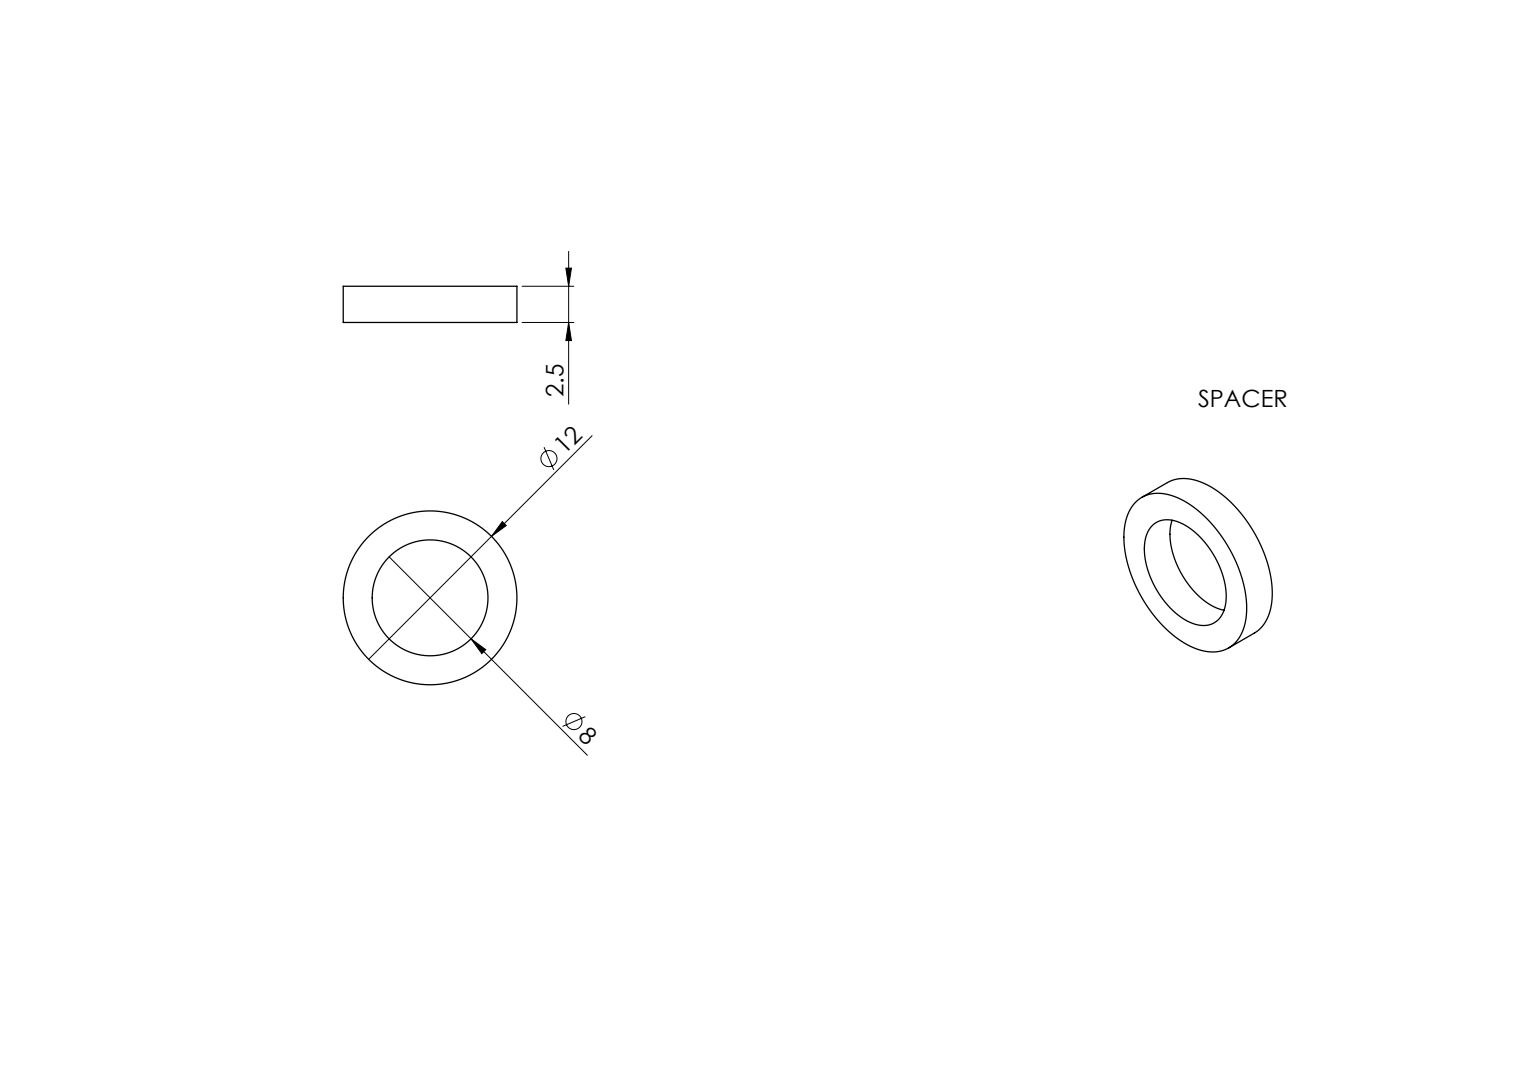
ISO-10303-21;
HEADER;
FILE_DESCRIPTION (('STEP AP214'),
    '1' );
FILE_NAME ('spacer.step',
    '2026-10-31T03:41:51',
    ( '' ),
    ( '' ),
    'SwSTEP 2.0',
    'SolidWorks 2026',
    '' );
FILE_SCHEMA (( 'AUTOMOTIVE_DESIGN' ));
ENDSEC;

DATA;
#19=FACE_OUTER_BOUND ( 'NONE', #11949, .T. ) ;
#42=CYLINDRICAL_SURFACE ( 'NONE', #425, 5.999999999999999112 ) ;
#89=ORIENTED_EDGE ( 'NONE', *, *, #1488, .F. ) ;
#125=PLANE ( 'NONE',  #1631 ) ;
#144=CARTESIAN_POINT ( 'NONE',  ( 0.000000000000000000, 0.000000000000000000, 3.895000000000000462 ) ) ;
#220=CIRCLE ( 'NONE', #8093, 5.999999999999999112 ) ;
#252=ADVANCED_FACE ( 'NONE', ( #6406, #6332 ), #7416, .F. ) ;
#355=ORIENTED_EDGE ( 'NONE', *, *, #8570, .F. ) ;
#402=ORIENTED_EDGE ( 'NONE', *, *, #5553, .T. ) ;
#425=AXIS2_PLACEMENT_3D ( 'NONE', #3589, #8419, #2592 ) ;
#542=PRODUCT_DEFINITION_CONTEXT ( 'detailed design', #8310, 'design' ) ;
#683=AXIS2_PLACEMENT_3D ( 'NONE', #4148, #11052, #7449 ) ;
#791=CARTESIAN_POINT ( 'NONE',  ( 4.000000000000000000, 4.898587196589412829E-16, 3.895000000000000462 ) ) ;
#805=AXIS2_PLACEMENT_3D ( 'NONE', #9265, #4731, #5810 ) ;
#1155=AXIS2_PLACEMENT_3D ( 'NONE', #2651, #6177, #5122 ) ;
#1175=CARTESIAN_POINT ( 'NONE',  ( -5.999999999999999112, 0.000000000000000000, 1.395000000000000462 ) ) ;
#1312=ORIENTED_EDGE ( 'NONE', *, *, #4480, .F. ) ;
#1357=DIRECTION ( 'NONE',  ( -0.000000000000000000, -0.000000000000000000, -1.000000000000000000 ) ) ;
#1376=AXIS2_PLACEMENT_3D ( 'NONE', #7353, #6187, #9640 ) ;
#1391=DIRECTION ( 'NONE',  ( 0.000000000000000000, 0.000000000000000000, -1.000000000000000000 ) ) ;
#1443=LINE ( 'NONE', #3512, #4366 ) ;
#1488=EDGE_CURVE ( 'NONE', #5963, #15052, #13663, .T. ) ;
#1631=AXIS2_PLACEMENT_3D ( 'NONE', #2376, #11890, #11748 ) ;
#1634=UNCERTAINTY_MEASURE_WITH_UNIT (LENGTH_MEASURE( 1.000000000000000082E-05 ), #6541, 'distance_accuracy_value', 'NONE');
#1705=SURFACE_STYLE_USAGE ( .BOTH. , #13375 ) ;
#1863=DIRECTION ( 'NONE',  ( -1.000000000000000000, 0.000000000000000000, 0.000000000000000000 ) ) ;
#1949=ADVANCED_FACE ( 'NONE', ( #3680, #12971 ), #125, .T. ) ;
#2053=DIRECTION ( 'NONE',  ( -0.000000000000000000, -0.000000000000000000, -1.000000000000000000 ) ) ;
#2054=EDGE_CURVE ( 'NONE', #3198, #8635, #12421, .T. ) ;
#2071=CARTESIAN_POINT ( 'NONE',  ( 0.000000000000000000, 0.000000000000000000, 3.895000000000000462 ) ) ;
#2078=VERTEX_POINT ( 'NONE', #9893 ) ;
#2095=EDGE_LOOP ( 'NONE', ( #8631, #14510 ) ) ;
#2126=( GEOMETRIC_REPRESENTATION_CONTEXT ( 3 ) GLOBAL_UNCERTAINTY_ASSIGNED_CONTEXT ( ( #1634 ) ) GLOBAL_UNIT_ASSIGNED_CONTEXT ( ( #6541, #8765, #3857 ) ) REPRESENTATION_CONTEXT ( 'NONE', 'WORKASPACE' ) );
#2208=ADVANCED_FACE ( 'NONE', ( #13742 ), #5387, .T. ) ;
#2376=CARTESIAN_POINT ( 'NONE',  ( 0.000000000000000000, 0.000000000000000000, 1.395000000000000462 ) ) ;
#2378=EDGE_CURVE ( 'NONE', #13028, #6156, #2757, .T. ) ;
#2438=DIRECTION ( 'NONE',  ( -1.000000000000000000, 0.000000000000000000, 0.000000000000000000 ) ) ;
#2443=CIRCLE ( 'NONE', #11027, 5.999999999999999112 ) ;
#2592=DIRECTION ( 'NONE',  ( -1.000000000000000000, 0.000000000000000000, 0.000000000000000000 ) ) ;
#2611=MECHANICAL_DESIGN_GEOMETRIC_PRESENTATION_REPRESENTATION('',(#9242),#10950);
#2651=CARTESIAN_POINT ( 'NONE',  ( 0.000000000000000000, 0.000000000000000000, 3.895000000000000462 ) ) ;
#2697=ORIENTED_EDGE ( 'NONE', *, *, #5601, .T. ) ;
#2757=CIRCLE ( 'NONE', #11337, 4.000000000000000000 ) ;
#2777=ORIENTED_EDGE ( 'NONE', *, *, #9895, .F. ) ;
#2831=CIRCLE ( 'NONE', #4804, 5.999999999999999112 ) ;
#2918=AXIS2_PLACEMENT_3D ( 'NONE', #11500, #15210, #6043 ) ;
#3163=CARTESIAN_POINT ( 'NONE',  ( 5.999999999999999112, 7.347880794884118750E-16, 3.895000000000000462 ) ) ;
#3198=VERTEX_POINT ( 'NONE', #11372 ) ;
#3220=CARTESIAN_POINT ( 'NONE',  ( 0.000000000000000000, 0.000000000000000000, 3.895000000000000462 ) ) ;
#3239=EDGE_LOOP ( 'NONE', ( #14240, #4911 ) ) ;
#3355=AXIS2_PLACEMENT_3D ( 'NONE', #5126, #7491, #14495 ) ;
#3480=AXIS2_PLACEMENT_3D ( 'NONE', #3220, #2053, #4220 ) ;
#3512=CARTESIAN_POINT ( 'NONE',  ( -5.999999999999999112, 0.000000000000000000, 3.895000000000000462 ) ) ;
#3589=CARTESIAN_POINT ( 'NONE',  ( 0.000000000000000000, 0.000000000000000000, 3.895000000000000462 ) ) ;
#3619=DIRECTION ( 'NONE',  ( -1.000000000000000000, 0.000000000000000000, 0.000000000000000000 ) ) ;
#3680=FACE_BOUND ( 'NONE', #3239, .T. ) ;
#3746=ORIENTED_EDGE ( 'NONE', *, *, #12567, .F. ) ;
#3857=( NAMED_UNIT ( * ) SI_UNIT ( $, .STERADIAN. ) SOLID_ANGLE_UNIT ( ) );
#4014=ADVANCED_FACE ( 'NONE', ( #19 ), #4890, .F. ) ;
#4057=PRODUCT_CONTEXT ( 'NONE', #14709, 'mechanical' ) ;
#4148=CARTESIAN_POINT ( 'NONE',  ( 0.000000000000000000, 0.000000000000000000, 3.895000000000000462 ) ) ;
#4220=DIRECTION ( 'NONE',  ( -1.000000000000000000, 0.000000000000000000, 0.000000000000000000 ) ) ;
#4282=SHAPE_DEFINITION_REPRESENTATION ( #5673, #13067 ) ;
#4366=VECTOR ( 'NONE', #1357, 1000.000000000000000 ) ;
#4480=EDGE_CURVE ( 'NONE', #2078, #3198, #7919, .T. ) ;
#4731=DIRECTION ( 'NONE',  ( -0.000000000000000000, -0.000000000000000000, -1.000000000000000000 ) ) ;
#4735=VECTOR ( 'NONE', #5693, 1000.000000000000000 ) ;
#4773=ORIENTED_EDGE ( 'NONE', *, *, #8992, .F. ) ;
#4804=AXIS2_PLACEMENT_3D ( 'NONE', #6467, #12381, #1863 ) ;
#4890=CYLINDRICAL_SURFACE ( 'NONE', #805, 4.000000000000000000 ) ;
#4911=ORIENTED_EDGE ( 'NONE', *, *, #2378, .F. ) ;
#5020=( NAMED_UNIT ( * ) PLANE_ANGLE_UNIT ( ) SI_UNIT ( $, .RADIAN. ) );
#5046=ORIENTED_EDGE ( 'NONE', *, *, #2378, .T. ) ;
#5079=CARTESIAN_POINT ( 'NONE',  ( 0.000000000000000000, 0.000000000000000000, 1.395000000000000462 ) ) ;
#5122=DIRECTION ( 'NONE',  ( -1.000000000000000000, 0.000000000000000000, -0.000000000000000000 ) ) ;
#5126=CARTESIAN_POINT ( 'NONE',  ( 0.000000000000000000, 0.000000000000000000, 3.895000000000000462 ) ) ;
#5322=CARTESIAN_POINT ( 'NONE',  ( 0.000000000000000000, 0.000000000000000000, 1.395000000000000462 ) ) ;
#5357=DIRECTION ( 'NONE',  ( -0.000000000000000000, -0.000000000000000000, -1.000000000000000000 ) ) ;
#5387=CYLINDRICAL_SURFACE ( 'NONE', #3480, 5.999999999999999112 ) ;
#5553=EDGE_CURVE ( 'NONE', #8635, #3198, #220, .T. ) ;
#5601=EDGE_CURVE ( 'NONE', #2078, #6712, #2443, .T. ) ;
#5668=DIRECTION ( 'NONE',  ( -0.000000000000000000, -0.000000000000000000, -1.000000000000000000 ) ) ;
#5673=PRODUCT_DEFINITION_SHAPE ( 'NONE', 'NONE',  #11139 ) ;
#5692=DIRECTION ( 'NONE',  ( -1.000000000000000000, 0.000000000000000000, 0.000000000000000000 ) ) ;
#5693=DIRECTION ( 'NONE',  ( -0.000000000000000000, -0.000000000000000000, -1.000000000000000000 ) ) ;
#5743=CARTESIAN_POINT ( 'NONE',  ( -4.000000000000000000, 0.000000000000000000, 1.395000000000000462 ) ) ;
#5810=DIRECTION ( 'NONE',  ( -1.000000000000000000, 0.000000000000000000, 0.000000000000000000 ) ) ;
#5868=ORIENTED_EDGE ( 'NONE', *, *, #9895, .T. ) ;
#5963=VERTEX_POINT ( 'NONE', #7376 ) ;
#6043=DIRECTION ( 'NONE',  ( -1.000000000000000000, 0.000000000000000000, 0.000000000000000000 ) ) ;
#6141=CYLINDRICAL_SURFACE ( 'NONE', #683, 4.000000000000000000 ) ;
#6156=VERTEX_POINT ( 'NONE', #5743 ) ;
#6177=DIRECTION ( 'NONE',  ( 0.000000000000000000, 0.000000000000000000, -1.000000000000000000 ) ) ;
#6187=DIRECTION ( 'NONE',  ( 0.000000000000000000, 0.000000000000000000, 1.000000000000000000 ) ) ;
#6249=( GEOMETRIC_REPRESENTATION_CONTEXT ( 3 ) GLOBAL_UNCERTAINTY_ASSIGNED_CONTEXT ( ( #11534 ) ) GLOBAL_UNIT_ASSIGNED_CONTEXT ( ( #14041, #10436, #7129 ) ) REPRESENTATION_CONTEXT ( 'NONE', 'WORKASPACE' ) );
#6332=FACE_OUTER_BOUND ( 'NONE', #14476, .T. ) ;
#6406=FACE_BOUND ( 'NONE', #2095, .T. ) ;
#6467=CARTESIAN_POINT ( 'NONE',  ( 0.000000000000000000, 0.000000000000000000, 3.895000000000000462 ) ) ;
#6541=( LENGTH_UNIT ( ) NAMED_UNIT ( * ) SI_UNIT ( .MILLI., .METRE. ) );
#6712=VERTEX_POINT ( 'NONE', #7172 ) ;
#6966=CARTESIAN_POINT ( 'NONE',  ( 0.000000000000000000, 0.000000000000000000, 1.395000000000000462 ) ) ;
#7035=AXIS2_PLACEMENT_3D ( 'NONE', #144, #1391, #3619 ) ;
#7040=ADVANCED_FACE ( 'NONE', ( #8513 ), #6141, .F. ) ;
#7129=( NAMED_UNIT ( * ) SI_UNIT ( $, .STERADIAN. ) SOLID_ANGLE_UNIT ( ) );
#7172=CARTESIAN_POINT ( 'NONE',  ( -5.999999999999999112, 0.000000000000000000, 3.895000000000000462 ) ) ;
#7216=CLOSED_SHELL ( 'NONE', ( #4014, #2208, #9609, #252, #1949, #7040 ) ) ;
#7282=CIRCLE ( 'NONE', #3355, 4.000000000000000000 ) ;
#7289=EDGE_CURVE ( 'NONE', #6156, #13028, #8799, .T. ) ;
#7346=ORIENTED_EDGE ( 'NONE', *, *, #2054, .T. ) ;
#7353=CARTESIAN_POINT ( 'NONE',  ( 0.000000000000000000, 0.000000000000000000, 0.000000000000000000 ) ) ;
#7376=CARTESIAN_POINT ( 'NONE',  ( -4.000000000000000000, 0.000000000000000000, 3.895000000000000462 ) ) ;
#7416=PLANE ( 'NONE',  #1155 ) ;
#7449=DIRECTION ( 'NONE',  ( -1.000000000000000000, 0.000000000000000000, 0.000000000000000000 ) ) ;
#7450=DIRECTION ( 'NONE',  ( 0.000000000000000000, 0.000000000000000000, -1.000000000000000000 ) ) ;
#7491=DIRECTION ( 'NONE',  ( 0.000000000000000000, 0.000000000000000000, -1.000000000000000000 ) ) ;
#7623=FILL_AREA_STYLE ('',( #8842 ) ) ;
#7687=DIRECTION ( 'NONE',  ( 0.000000000000000000, 0.000000000000000000, -1.000000000000000000 ) ) ;
#7693=SHAPE_REPRESENTATION_RELATIONSHIP ( 'NONE' , 'NONE' ,  #13067, #8180 ) ;
#7722=STYLED_ITEM('',(#15265),#8383);
#7901=EDGE_LOOP ( 'NONE', ( #9151, #8082, #14292, #9298 ) ) ;
#7919=LINE ( 'NONE', #3163, #4735 ) ;
#8000=EDGE_LOOP ( 'NONE', ( #355, #89, #5868, #8665 ) ) ;
#8082=ORIENTED_EDGE ( 'NONE', *, *, #4480, .T. ) ;
#8093=AXIS2_PLACEMENT_3D ( 'NONE', #5322, #14694, #8837 ) ;
#8180=ADVANCED_BREP_SHAPE_REPRESENTATION ( '', ( #8383, #1376 ), #2126 ) ;
#8310=APPLICATION_CONTEXT ( 'automotive_design' ) ;
#8367=EDGE_LOOP ( 'NONE', ( #1312, #2697, #12223, #12430 ) ) ;
#8383=MANIFOLD_SOLID_BREP ( 'Boss-Extrude1', #7216 ) ;
#8419=DIRECTION ( 'NONE',  ( -0.000000000000000000, -0.000000000000000000, -1.000000000000000000 ) ) ;
#8513=FACE_OUTER_BOUND ( 'NONE', #8000, .T. ) ;
#8541=( LENGTH_UNIT ( ) NAMED_UNIT ( * ) SI_UNIT ( .MILLI., .METRE. ) );
#8570=EDGE_CURVE ( 'NONE', #15052, #13028, #14866, .T. ) ;
#8631=ORIENTED_EDGE ( 'NONE', *, *, #1488, .T. ) ;
#8635=VERTEX_POINT ( 'NONE', #1175 ) ;
#8665=ORIENTED_EDGE ( 'NONE', *, *, #7289, .T. ) ;
#8765=( NAMED_UNIT ( * ) PLANE_ANGLE_UNIT ( ) SI_UNIT ( $, .RADIAN. ) );
#8799=CIRCLE ( 'NONE', #2918, 4.000000000000000000 ) ;
#8837=DIRECTION ( 'NONE',  ( -1.000000000000000000, 0.000000000000000000, 0.000000000000000000 ) ) ;
#8842=FILL_AREA_STYLE_COLOUR ( '', #14152 ) ;
#8846=CARTESIAN_POINT ( 'NONE',  ( 4.000000000000000000, 4.898587196589412829E-16, 1.395000000000000462 ) ) ;
#8945=MECHANICAL_DESIGN_GEOMETRIC_PRESENTATION_REPRESENTATION('',(#7722),#6249);
#8992=EDGE_CURVE ( 'NONE', #6712, #2078, #2831, .T. ) ;
#9151=ORIENTED_EDGE ( 'NONE', *, *, #8992, .T. ) ;
#9242=STYLED_ITEM ( 'NONE', ( #13535 ), #8180 ) ;
#9265=CARTESIAN_POINT ( 'NONE',  ( 0.000000000000000000, 0.000000000000000000, 3.895000000000000462 ) ) ;
#9298=ORIENTED_EDGE ( 'NONE', *, *, #9550, .F. ) ;
#9550=EDGE_CURVE ( 'NONE', #6712, #8635, #1443, .T. ) ;
#9609=ADVANCED_FACE ( 'NONE', ( #11804 ), #42, .T. ) ;
#9640=DIRECTION ( 'NONE',  ( 1.000000000000000000, 0.000000000000000000, 0.000000000000000000 ) ) ;
#9893=CARTESIAN_POINT ( 'NONE',  ( 5.999999999999999112, 7.347880794884118750E-16, 3.895000000000000462 ) ) ;
#9895=EDGE_CURVE ( 'NONE', #5963, #6156, #10272, .T. ) ;
#9936=VECTOR ( 'NONE', #5357, 1000.000000000000000 ) ;
#10272=LINE ( 'NONE', #13573, #12224 ) ;
#10436=( NAMED_UNIT ( * ) PLANE_ANGLE_UNIT ( ) SI_UNIT ( $, .RADIAN. ) );
#10950=( GEOMETRIC_REPRESENTATION_CONTEXT ( 3 ) GLOBAL_UNCERTAINTY_ASSIGNED_CONTEXT ( ( #13304 ) ) GLOBAL_UNIT_ASSIGNED_CONTEXT ( ( #8541, #5020, #14390 ) ) REPRESENTATION_CONTEXT ( 'NONE', 'WORKASPACE' ) );
#11027=AXIS2_PLACEMENT_3D ( 'NONE', #2071, #7687, #5692 ) ;
#11052=DIRECTION ( 'NONE',  ( -0.000000000000000000, -0.000000000000000000, -1.000000000000000000 ) ) ;
#11139=PRODUCT_DEFINITION ( 'UNKNOWN', '', #12636, #542 ) ;
#11337=AXIS2_PLACEMENT_3D ( 'NONE', #6966, #15211, #2438 ) ;
#11372=CARTESIAN_POINT ( 'NONE',  ( 5.999999999999999112, 7.347880794884118750E-16, 1.395000000000000462 ) ) ;
#11500=CARTESIAN_POINT ( 'NONE',  ( 0.000000000000000000, 0.000000000000000000, 1.395000000000000462 ) ) ;
#11534=UNCERTAINTY_MEASURE_WITH_UNIT (LENGTH_MEASURE( 1.000000000000000082E-05 ), #14041, 'distance_accuracy_value', 'NONE');
#11748=DIRECTION ( 'NONE',  ( -1.000000000000000000, 0.000000000000000000, -0.000000000000000000 ) ) ;
#11804=FACE_OUTER_BOUND ( 'NONE', #8367, .T. ) ;
#11890=DIRECTION ( 'NONE',  ( 0.000000000000000000, 0.000000000000000000, -1.000000000000000000 ) ) ;
#11949=EDGE_LOOP ( 'NONE', ( #3746, #12356, #5046, #2777 ) ) ;
#12223=ORIENTED_EDGE ( 'NONE', *, *, #9550, .T. ) ;
#12224=VECTOR ( 'NONE', #5668, 1000.000000000000000 ) ;
#12302=ORIENTED_EDGE ( 'NONE', *, *, #5601, .F. ) ;
#12356=ORIENTED_EDGE ( 'NONE', *, *, #8570, .T. ) ;
#12381=DIRECTION ( 'NONE',  ( 0.000000000000000000, 0.000000000000000000, -1.000000000000000000 ) ) ;
#12421=CIRCLE ( 'NONE', #14652, 5.999999999999999112 ) ;
#12430=ORIENTED_EDGE ( 'NONE', *, *, #2054, .F. ) ;
#12533=EDGE_LOOP ( 'NONE', ( #402, #7346 ) ) ;
#12567=EDGE_CURVE ( 'NONE', #15052, #5963, #7282, .T. ) ;
#12636=PRODUCT_DEFINITION_FORMATION_WITH_SPECIFIED_SOURCE ( 'ANY', '', #14394, .NOT_KNOWN. ) ;
#12971=FACE_OUTER_BOUND ( 'NONE', #12533, .T. ) ;
#13028=VERTEX_POINT ( 'NONE', #8846 ) ;
#13067=SHAPE_REPRESENTATION ( 'spacer', ( #1376 ), #2126 ) ;
#13296=SURFACE_STYLE_FILL_AREA ( #7623 ) ;
#13304=UNCERTAINTY_MEASURE_WITH_UNIT (LENGTH_MEASURE( 1.000000000000000082E-05 ), #8541, 'distance_accuracy_value', 'NONE');
#13350=DIRECTION ( 'NONE',  ( -1.000000000000000000, 0.000000000000000000, 0.000000000000000000 ) ) ;
#13375=SURFACE_SIDE_STYLE ('',( #13296 ) ) ;
#13535=PRESENTATION_STYLE_ASSIGNMENT (( #1705 ) ) ;
#13573=CARTESIAN_POINT ( 'NONE',  ( -4.000000000000000000, 0.000000000000000000, 3.895000000000000462 ) ) ;
#13574=CARTESIAN_POINT ( 'NONE',  ( 4.000000000000000000, 4.898587196589412829E-16, 3.895000000000000462 ) ) ;
#13663=CIRCLE ( 'NONE', #7035, 4.000000000000000000 ) ;
#13742=FACE_OUTER_BOUND ( 'NONE', #7901, .T. ) ;
#14041=( LENGTH_UNIT ( ) NAMED_UNIT ( * ) SI_UNIT ( .MILLI., .METRE. ) );
#14152=COLOUR_RGB ( '',0.8941176470588234615, 0.8941176470588234615, 0.8941176470588234615 ) ;
#14240=ORIENTED_EDGE ( 'NONE', *, *, #7289, .F. ) ;
#14292=ORIENTED_EDGE ( 'NONE', *, *, #5553, .F. ) ;
#14390=( NAMED_UNIT ( * ) SI_UNIT ( $, .STERADIAN. ) SOLID_ANGLE_UNIT ( ) );
#14394=PRODUCT ( 'spacer', 'spacer', '', ( #4057 ) ) ;
#14476=EDGE_LOOP ( 'NONE', ( #4773, #12302 ) ) ;
#14495=DIRECTION ( 'NONE',  ( -1.000000000000000000, 0.000000000000000000, 0.000000000000000000 ) ) ;
#14510=ORIENTED_EDGE ( 'NONE', *, *, #12567, .T. ) ;
#14652=AXIS2_PLACEMENT_3D ( 'NONE', #5079, #7450, #13350 ) ;
#14694=DIRECTION ( 'NONE',  ( 0.000000000000000000, 0.000000000000000000, -1.000000000000000000 ) ) ;
#14709=APPLICATION_CONTEXT ( 'automotive_design' ) ;
#14866=LINE ( 'NONE', #791, #9936 ) ;
#15052=VERTEX_POINT ( 'NONE', #13574 ) ;
#15210=DIRECTION ( 'NONE',  ( 0.000000000000000000, 0.000000000000000000, -1.000000000000000000 ) ) ;
#15211=DIRECTION ( 'NONE',  ( 0.000000000000000000, 0.000000000000000000, -1.000000000000000000 ) ) ;
#15259=COLOUR_RGB('Sky Blue',0.24,0.69,0.87);
#15260=FILL_AREA_STYLE_COLOUR('',#15259);
#15261=FILL_AREA_STYLE('',(#15260));
#15262=SURFACE_STYLE_FILL_AREA(#15261);
#15263=SURFACE_SIDE_STYLE('',(#15262));
#15264=SURFACE_STYLE_USAGE(.BOTH.,#15263);
#15265=PRESENTATION_STYLE_ASSIGNMENT((#15264));
ENDSEC;
END-ISO-10303-21;
